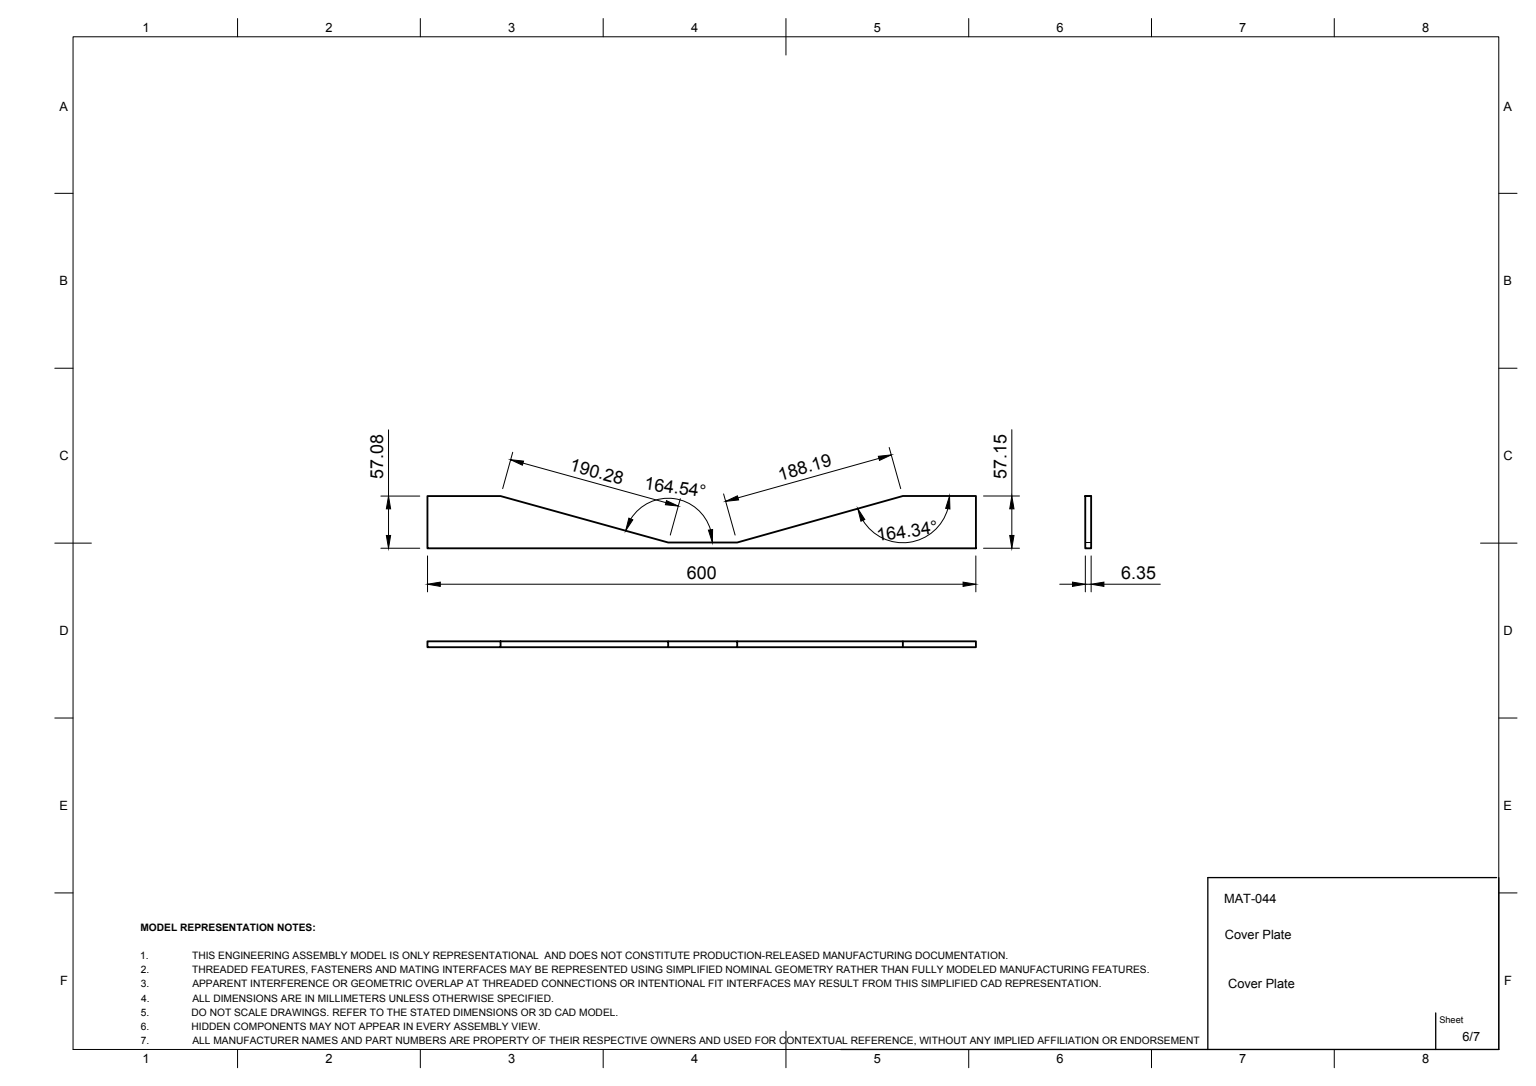
ISO-10303-21;
HEADER;
/* Generated by software containing ST-Developer
 * from STEP Tools, Inc. (www.steptools.com) 
 */

FILE_DESCRIPTION(
/* description */ ('STEP AP214'),
/* implementation_level */ '2;1');

FILE_NAME(
/* name */ 'Cover Plate.step',
/* time_stamp */ '2026-11-14T22:20:24-08:00',
/* author */ (''),
/* organization */ (''),
/* preprocessor_version */ 'ST-DEVELOPER v20.2',
/* originating_system */ 'Autodesk Translation Framework v15.17.0.0',
/* authorisation */ '');

FILE_SCHEMA (('AUTOMOTIVE_DESIGN { 1 0 10303 214 3 1 1 }'));
ENDSEC;

DATA;
#10=MECHANICAL_DESIGN_GEOMETRIC_PRESENTATION_REPRESENTATION('',(#84),#2794);
#74=SHAPE_REPRESENTATION_RELATIONSHIP('SRR','None',#2829,#79);
#79=ADVANCED_BREP_SHAPE_REPRESENTATION('',(#89),#2791);
#84=STYLED_ITEM('',(#2863),#89);
#89=MANIFOLD_SOLID_BREP('Body1',#1643);
#168=PLANE('',#1812);
#169=PLANE('',#1813);
#170=PLANE('',#1814);
#171=PLANE('',#1815);
#172=PLANE('',#1816);
#173=PLANE('',#1817);
#174=PLANE('',#1818);
#175=PLANE('',#1819);
#176=PLANE('',#1820);
#177=PLANE('',#1821);
#256=FACE_OUTER_BOUND('',#369,.T.);
#257=FACE_OUTER_BOUND('',#370,.T.);
#258=FACE_OUTER_BOUND('',#371,.T.);
#259=FACE_OUTER_BOUND('',#372,.T.);
#260=FACE_OUTER_BOUND('',#373,.T.);
#261=FACE_OUTER_BOUND('',#374,.T.);
#262=FACE_OUTER_BOUND('',#375,.T.);
#263=FACE_OUTER_BOUND('',#376,.T.);
#264=FACE_OUTER_BOUND('',#377,.T.);
#265=FACE_OUTER_BOUND('',#378,.T.);
#369=EDGE_LOOP('',(#1442,#1443,#1444,#1445));
#370=EDGE_LOOP('',(#1446,#1447,#1448,#1449));
#371=EDGE_LOOP('',(#1450,#1451,#1452,#1453));
#372=EDGE_LOOP('',(#1454,#1455,#1456,#1457));
#373=EDGE_LOOP('',(#1458,#1459,#1460,#1461));
#374=EDGE_LOOP('',(#1462,#1463,#1464,#1465));
#375=EDGE_LOOP('',(#1466,#1467,#1468,#1469));
#376=EDGE_LOOP('',(#1470,#1471,#1472,#1473));
#377=EDGE_LOOP('',(#1474,#1475,#1476,#1477,#1478,#1479,#1480,#1481));
#378=EDGE_LOOP('',(#1482,#1483,#1484,#1485,#1486,#1487,#1488,#1489));
#522=LINE('',#2673,#691);
#523=LINE('',#2675,#692);
#524=LINE('',#2677,#693);
#525=LINE('',#2678,#694);
#526=LINE('',#2681,#695);
#527=LINE('',#2683,#696);
#528=LINE('',#2684,#697);
#529=LINE('',#2687,#698);
#530=LINE('',#2689,#699);
#531=LINE('',#2690,#700);
#532=LINE('',#2693,#701);
#533=LINE('',#2695,#702);
#534=LINE('',#2696,#703);
#535=LINE('',#2699,#704);
#536=LINE('',#2701,#705);
#537=LINE('',#2702,#706);
#538=LINE('',#2705,#707);
#539=LINE('',#2707,#708);
#540=LINE('',#2708,#709);
#541=LINE('',#2711,#710);
#542=LINE('',#2713,#711);
#543=LINE('',#2714,#712);
#544=LINE('',#2716,#713);
#545=LINE('',#2717,#714);
#691=VECTOR('',#2207,1000.);
#692=VECTOR('',#2208,1000.);
#693=VECTOR('',#2209,1000.);
#694=VECTOR('',#2210,1000.);
#695=VECTOR('',#2213,1000.);
#696=VECTOR('',#2214,1000.);
#697=VECTOR('',#2215,1000.);
#698=VECTOR('',#2218,1000.);
#699=VECTOR('',#2219,1000.);
#700=VECTOR('',#2220,1000.);
#701=VECTOR('',#2223,1000.);
#702=VECTOR('',#2224,1000.);
#703=VECTOR('',#2225,1000.);
#704=VECTOR('',#2228,1000.);
#705=VECTOR('',#2229,1000.);
#706=VECTOR('',#2230,1000.);
#707=VECTOR('',#2233,1000.);
#708=VECTOR('',#2234,1000.);
#709=VECTOR('',#2235,1000.);
#710=VECTOR('',#2238,1000.);
#711=VECTOR('',#2239,1000.);
#712=VECTOR('',#2240,1000.);
#713=VECTOR('',#2243,1000.);
#714=VECTOR('',#2244,1000.);
#871=VERTEX_POINT('',#2671);
#872=VERTEX_POINT('',#2672);
#873=VERTEX_POINT('',#2674);
#874=VERTEX_POINT('',#2676);
#875=VERTEX_POINT('',#2680);
#876=VERTEX_POINT('',#2682);
#877=VERTEX_POINT('',#2686);
#878=VERTEX_POINT('',#2688);
#879=VERTEX_POINT('',#2692);
#880=VERTEX_POINT('',#2694);
#881=VERTEX_POINT('',#2698);
#882=VERTEX_POINT('',#2700);
#883=VERTEX_POINT('',#2704);
#884=VERTEX_POINT('',#2706);
#885=VERTEX_POINT('',#2710);
#886=VERTEX_POINT('',#2712);
#1066=EDGE_CURVE('',#871,#872,#522,.T.);
#1067=EDGE_CURVE('',#873,#872,#523,.T.);
#1068=EDGE_CURVE('',#874,#873,#524,.T.);
#1069=EDGE_CURVE('',#874,#871,#525,.T.);
#1070=EDGE_CURVE('',#872,#875,#526,.T.);
#1071=EDGE_CURVE('',#876,#875,#527,.T.);
#1072=EDGE_CURVE('',#873,#876,#528,.T.);
#1073=EDGE_CURVE('',#875,#877,#529,.T.);
#1074=EDGE_CURVE('',#878,#877,#530,.T.);
#1075=EDGE_CURVE('',#876,#878,#531,.T.);
#1076=EDGE_CURVE('',#877,#879,#532,.T.);
#1077=EDGE_CURVE('',#880,#879,#533,.T.);
#1078=EDGE_CURVE('',#878,#880,#534,.T.);
#1079=EDGE_CURVE('',#879,#881,#535,.T.);
#1080=EDGE_CURVE('',#882,#881,#536,.T.);
#1081=EDGE_CURVE('',#880,#882,#537,.T.);
#1082=EDGE_CURVE('',#881,#883,#538,.T.);
#1083=EDGE_CURVE('',#884,#883,#539,.T.);
#1084=EDGE_CURVE('',#882,#884,#540,.T.);
#1085=EDGE_CURVE('',#883,#885,#541,.T.);
#1086=EDGE_CURVE('',#886,#885,#542,.T.);
#1087=EDGE_CURVE('',#884,#886,#543,.T.);
#1088=EDGE_CURVE('',#885,#871,#544,.T.);
#1089=EDGE_CURVE('',#886,#874,#545,.T.);
#1442=ORIENTED_EDGE('',*,*,#1066,.T.);
#1443=ORIENTED_EDGE('',*,*,#1067,.F.);
#1444=ORIENTED_EDGE('',*,*,#1068,.F.);
#1445=ORIENTED_EDGE('',*,*,#1069,.T.);
#1446=ORIENTED_EDGE('',*,*,#1070,.T.);
#1447=ORIENTED_EDGE('',*,*,#1071,.F.);
#1448=ORIENTED_EDGE('',*,*,#1072,.F.);
#1449=ORIENTED_EDGE('',*,*,#1067,.T.);
#1450=ORIENTED_EDGE('',*,*,#1073,.T.);
#1451=ORIENTED_EDGE('',*,*,#1074,.F.);
#1452=ORIENTED_EDGE('',*,*,#1075,.F.);
#1453=ORIENTED_EDGE('',*,*,#1071,.T.);
#1454=ORIENTED_EDGE('',*,*,#1076,.T.);
#1455=ORIENTED_EDGE('',*,*,#1077,.F.);
#1456=ORIENTED_EDGE('',*,*,#1078,.F.);
#1457=ORIENTED_EDGE('',*,*,#1074,.T.);
#1458=ORIENTED_EDGE('',*,*,#1079,.T.);
#1459=ORIENTED_EDGE('',*,*,#1080,.F.);
#1460=ORIENTED_EDGE('',*,*,#1081,.F.);
#1461=ORIENTED_EDGE('',*,*,#1077,.T.);
#1462=ORIENTED_EDGE('',*,*,#1082,.T.);
#1463=ORIENTED_EDGE('',*,*,#1083,.F.);
#1464=ORIENTED_EDGE('',*,*,#1084,.F.);
#1465=ORIENTED_EDGE('',*,*,#1080,.T.);
#1466=ORIENTED_EDGE('',*,*,#1085,.T.);
#1467=ORIENTED_EDGE('',*,*,#1086,.F.);
#1468=ORIENTED_EDGE('',*,*,#1087,.F.);
#1469=ORIENTED_EDGE('',*,*,#1083,.T.);
#1470=ORIENTED_EDGE('',*,*,#1088,.T.);
#1471=ORIENTED_EDGE('',*,*,#1069,.F.);
#1472=ORIENTED_EDGE('',*,*,#1089,.F.);
#1473=ORIENTED_EDGE('',*,*,#1086,.T.);
#1474=ORIENTED_EDGE('',*,*,#1068,.T.);
#1475=ORIENTED_EDGE('',*,*,#1072,.T.);
#1476=ORIENTED_EDGE('',*,*,#1075,.T.);
#1477=ORIENTED_EDGE('',*,*,#1078,.T.);
#1478=ORIENTED_EDGE('',*,*,#1081,.T.);
#1479=ORIENTED_EDGE('',*,*,#1084,.T.);
#1480=ORIENTED_EDGE('',*,*,#1087,.T.);
#1481=ORIENTED_EDGE('',*,*,#1089,.T.);
#1482=ORIENTED_EDGE('',*,*,#1066,.F.);
#1483=ORIENTED_EDGE('',*,*,#1088,.F.);
#1484=ORIENTED_EDGE('',*,*,#1085,.F.);
#1485=ORIENTED_EDGE('',*,*,#1082,.F.);
#1486=ORIENTED_EDGE('',*,*,#1079,.F.);
#1487=ORIENTED_EDGE('',*,*,#1076,.F.);
#1488=ORIENTED_EDGE('',*,*,#1073,.F.);
#1489=ORIENTED_EDGE('',*,*,#1070,.F.);
#1620=ADVANCED_FACE('',(#256),#168,.F.);
#1621=ADVANCED_FACE('',(#257),#169,.F.);
#1622=ADVANCED_FACE('',(#258),#170,.F.);
#1623=ADVANCED_FACE('',(#259),#171,.F.);
#1624=ADVANCED_FACE('',(#260),#172,.F.);
#1625=ADVANCED_FACE('',(#261),#173,.F.);
#1626=ADVANCED_FACE('',(#262),#174,.F.);
#1627=ADVANCED_FACE('',(#263),#175,.F.);
#1628=ADVANCED_FACE('',(#264),#176,.F.);
#1629=ADVANCED_FACE('',(#265),#177,.T.);
#1643=CLOSED_SHELL('',(#1620,#1621,#1622,#1623,#1624,#1625,#1626,#1627,
#1628,#1629));
#1811=AXIS2_PLACEMENT_3D('',#2669,#2203,#2204);
#1812=AXIS2_PLACEMENT_3D('',#2670,#2205,#2206);
#1813=AXIS2_PLACEMENT_3D('',#2679,#2211,#2212);
#1814=AXIS2_PLACEMENT_3D('',#2685,#2216,#2217);
#1815=AXIS2_PLACEMENT_3D('',#2691,#2221,#2222);
#1816=AXIS2_PLACEMENT_3D('',#2697,#2226,#2227);
#1817=AXIS2_PLACEMENT_3D('',#2703,#2231,#2232);
#1818=AXIS2_PLACEMENT_3D('',#2709,#2236,#2237);
#1819=AXIS2_PLACEMENT_3D('',#2715,#2241,#2242);
#1820=AXIS2_PLACEMENT_3D('',#2718,#2245,#2246);
#1821=AXIS2_PLACEMENT_3D('',#2719,#2247,#2248);
#2203=DIRECTION('axis',(0.,0.,1.));
#2204=DIRECTION('refdir',(1.,0.,0.));
#2205=DIRECTION('center_axis',(0.,1.,0.));
#2206=DIRECTION('ref_axis',(0.,0.,1.));
#2207=DIRECTION('',(1.,0.,0.));
#2208=DIRECTION('',(0.,0.,-1.));
#2209=DIRECTION('',(1.,0.,0.));
#2210=DIRECTION('',(0.,0.,-1.));
#2211=DIRECTION('center_axis',(-1.,0.,0.));
#2212=DIRECTION('ref_axis',(0.,0.,1.));
#2213=DIRECTION('',(0.,1.,0.));
#2214=DIRECTION('',(0.,0.,-1.));
#2215=DIRECTION('',(0.,1.,0.));
#2216=DIRECTION('center_axis',(0.,-1.,0.));
#2217=DIRECTION('ref_axis',(0.,0.,-1.));
#2218=DIRECTION('',(-1.,0.,0.));
#2219=DIRECTION('',(0.,0.,-1.));
#2220=DIRECTION('',(-1.,0.,0.));
#2221=DIRECTION('center_axis',(0.266610574094054,-0.963804337913686,0.));
#2222=DIRECTION('ref_axis',(0.963804337913686,0.266610574094054,0.));
#2223=DIRECTION('',(-0.963804337913686,-0.266610574094054,0.));
#2224=DIRECTION('',(0.,0.,-1.));
#2225=DIRECTION('',(-0.963804337913686,-0.266610574094054,0.));
#2226=DIRECTION('center_axis',(0.,-1.,0.));
#2227=DIRECTION('ref_axis',(0.,0.,-1.));
#2228=DIRECTION('',(-1.,0.,0.));
#2229=DIRECTION('',(0.,0.,-1.));
#2230=DIRECTION('',(-1.,0.,0.));
#2231=DIRECTION('center_axis',(-0.26994323774403,-0.962876237320389,0.));
#2232=DIRECTION('ref_axis',(0.962876237320389,-0.26994323774403,0.));
#2233=DIRECTION('',(-0.962876237320389,0.26994323774403,0.));
#2234=DIRECTION('',(0.,0.,-1.));
#2235=DIRECTION('',(-0.962876237320389,0.26994323774403,0.));
#2236=DIRECTION('center_axis',(0.,-1.,0.));
#2237=DIRECTION('ref_axis',(0.,0.,-1.));
#2238=DIRECTION('',(-1.,0.,0.));
#2239=DIRECTION('',(0.,0.,-1.));
#2240=DIRECTION('',(-1.,0.,0.));
#2241=DIRECTION('center_axis',(1.,0.,0.));
#2242=DIRECTION('ref_axis',(0.,0.,-1.));
#2243=DIRECTION('',(0.,-1.,0.));
#2244=DIRECTION('',(0.,-1.,0.));
#2245=DIRECTION('center_axis',(0.,0.,-1.));
#2246=DIRECTION('ref_axis',(-1.,0.,0.));
#2247=DIRECTION('center_axis',(0.,0.,-1.));
#2248=DIRECTION('ref_axis',(-1.,0.,0.));
#2669=CARTESIAN_POINT('',(0.,0.,0.));
#2670=CARTESIAN_POINT('Origin',(600.,0.,6.35000000000008));
#2671=CARTESIAN_POINT('',(0.,0.,0.));
#2672=CARTESIAN_POINT('',(600.,0.,0.));
#2673=CARTESIAN_POINT('',(600.,0.,0.));
#2674=CARTESIAN_POINT('',(600.,0.,6.35000000000008));
#2675=CARTESIAN_POINT('',(600.,0.,6.35000000000008));
#2676=CARTESIAN_POINT('',(0.,0.,6.35000000000008));
#2677=CARTESIAN_POINT('',(600.,0.,6.35000000000008));
#2678=CARTESIAN_POINT('',(0.,0.,6.35000000000008));
#2679=CARTESIAN_POINT('Origin',(600.,57.0813206381415,6.35000000000008));
#2680=CARTESIAN_POINT('',(600.,57.0813206381415,0.));
#2681=CARTESIAN_POINT('',(600.,57.0813206381415,0.));
#2682=CARTESIAN_POINT('',(600.,57.0813206381415,6.35000000000008));
#2683=CARTESIAN_POINT('',(600.,57.0813206381415,6.35000000000008));
#2684=CARTESIAN_POINT('',(600.,57.0813206381415,6.35000000000008));
#2685=CARTESIAN_POINT('Origin',(520.009455205772,57.0813206381415,6.35000000000008));
#2686=CARTESIAN_POINT('',(520.009455205772,57.0813206381415,0.));
#2687=CARTESIAN_POINT('',(520.009455205772,57.0813206381415,0.));
#2688=CARTESIAN_POINT('',(520.009455205772,57.0813206381415,6.35000000000008));
#2689=CARTESIAN_POINT('',(520.009455205772,57.0813206381415,6.35000000000008));
#2690=CARTESIAN_POINT('',(520.009455205772,57.0813206381415,6.35000000000008));
#2691=CARTESIAN_POINT('Origin',(336.61437770265,6.34999999999989,6.35000000000008));
#2692=CARTESIAN_POINT('',(336.61437770265,6.34999999999989,0.));
#2693=CARTESIAN_POINT('',(336.61437770265,6.34999999999989,0.));
#2694=CARTESIAN_POINT('',(336.61437770265,6.34999999999989,6.35000000000008));
#2695=CARTESIAN_POINT('',(336.61437770265,6.34999999999989,6.35000000000008));
#2696=CARTESIAN_POINT('',(336.61437770265,6.34999999999989,6.35000000000008));
#2697=CARTESIAN_POINT('Origin',(261.137671718493,6.34999999999989,6.35000000000008));
#2698=CARTESIAN_POINT('',(261.137671718493,6.34999999999989,0.));
#2699=CARTESIAN_POINT('',(261.137671718493,6.34999999999989,0.));
#2700=CARTESIAN_POINT('',(261.137671718493,6.34999999999989,6.35000000000008));
#2701=CARTESIAN_POINT('',(261.137671718493,6.34999999999989,6.35000000000008));
#2702=CARTESIAN_POINT('',(261.137671718493,6.34999999999989,6.35000000000008));
#2703=CARTESIAN_POINT('Origin',(79.9361966800339,57.1499999999999,6.35000000000008));
#2704=CARTESIAN_POINT('',(79.9361966800339,57.1499999999999,0.));
#2705=CARTESIAN_POINT('',(79.9361966800339,57.1499999999999,0.));
#2706=CARTESIAN_POINT('',(79.9361966800339,57.1499999999999,6.35000000000008));
#2707=CARTESIAN_POINT('',(79.9361966800339,57.1499999999999,6.35000000000008));
#2708=CARTESIAN_POINT('',(79.9361966800339,57.1499999999999,6.35000000000008));
#2709=CARTESIAN_POINT('Origin',(0.,57.1499999999999,6.35000000000008));
#2710=CARTESIAN_POINT('',(0.,57.1499999999999,0.));
#2711=CARTESIAN_POINT('',(0.,57.1499999999999,0.));
#2712=CARTESIAN_POINT('',(0.,57.1499999999999,6.35000000000008));
#2713=CARTESIAN_POINT('',(0.,57.1499999999999,6.35000000000008));
#2714=CARTESIAN_POINT('',(0.,57.1499999999999,6.35000000000008));
#2715=CARTESIAN_POINT('Origin',(0.,0.,6.35000000000008));
#2716=CARTESIAN_POINT('',(0.,0.,0.));
#2717=CARTESIAN_POINT('',(0.,0.,6.35000000000008));
#2718=CARTESIAN_POINT('Origin',(0.,0.,6.35000000000008));
#2719=CARTESIAN_POINT('Origin',(0.,0.,0.));
#2784=UNCERTAINTY_MEASURE_WITH_UNIT(LENGTH_MEASURE(0.01),#2795,
'DISTANCE_ACCURACY_VALUE',
'Maximum model space distance between geometric entities at asserted c
onnectivities');
#2787=UNCERTAINTY_MEASURE_WITH_UNIT(LENGTH_MEASURE(0.01),#2795,
'DISTANCE_ACCURACY_VALUE',
'Maximum model space distance between geometric entities at asserted c
onnectivities');
#2791=(
GEOMETRIC_REPRESENTATION_CONTEXT(3)
GLOBAL_UNCERTAINTY_ASSIGNED_CONTEXT((#2784))
GLOBAL_UNIT_ASSIGNED_CONTEXT((#2795,#2797,#2798))
REPRESENTATION_CONTEXT('','3D')
);
#2794=(
GEOMETRIC_REPRESENTATION_CONTEXT(3)
GLOBAL_UNCERTAINTY_ASSIGNED_CONTEXT((#2787))
GLOBAL_UNIT_ASSIGNED_CONTEXT((#2795,#2797,#2798))
REPRESENTATION_CONTEXT('','3D')
);
#2795=(
LENGTH_UNIT()
NAMED_UNIT(*)
SI_UNIT(.MILLI.,.METRE.)
);
#2797=(
NAMED_UNIT(*)
PLANE_ANGLE_UNIT()
SI_UNIT($,.RADIAN.)
);
#2798=(
NAMED_UNIT(*)
SI_UNIT($,.STERADIAN.)
SOLID_ANGLE_UNIT()
);
#2802=SHAPE_DEFINITION_REPRESENTATION(#2808,#2829);
#2808=PRODUCT_DEFINITION_SHAPE('',$,#2836);
#2829=SHAPE_REPRESENTATION('',(#1811),#2791);
#2832=PRODUCT_DEFINITION_CONTEXT('part definition',#2852,'design');
#2836=PRODUCT_DEFINITION('Cover Plate','Cover Plate',#2842,#2832);
#2842=PRODUCT_DEFINITION_FORMATION('',$,#2857);
#2852=APPLICATION_CONTEXT(
'Core Data for Automotive Mechanical Design Process');
#2853=PRODUCT_CONTEXT('part definition',#2852,'mechanical');
#2857=PRODUCT('Cover Plate','Cover Plate',$,(#2853));
#2863=PRESENTATION_STYLE_ASSIGNMENT((#2867));
#2867=SURFACE_STYLE_USAGE(.BOTH.,#2871);
#2871=SURFACE_SIDE_STYLE('',(#2875));
#2875=SURFACE_STYLE_FILL_AREA(#2879);
#2879=FILL_AREA_STYLE('Opaque(227,224,212)',(#2883));
#2883=FILL_AREA_STYLE_COLOUR('Opaque(227,224,212)',#2887);
#2887=COLOUR_RGB('Opaque(227,224,212)',0.890196078431372,0.87843137254902,
0.831372549019608);
ENDSEC;
END-ISO-10303-21;
